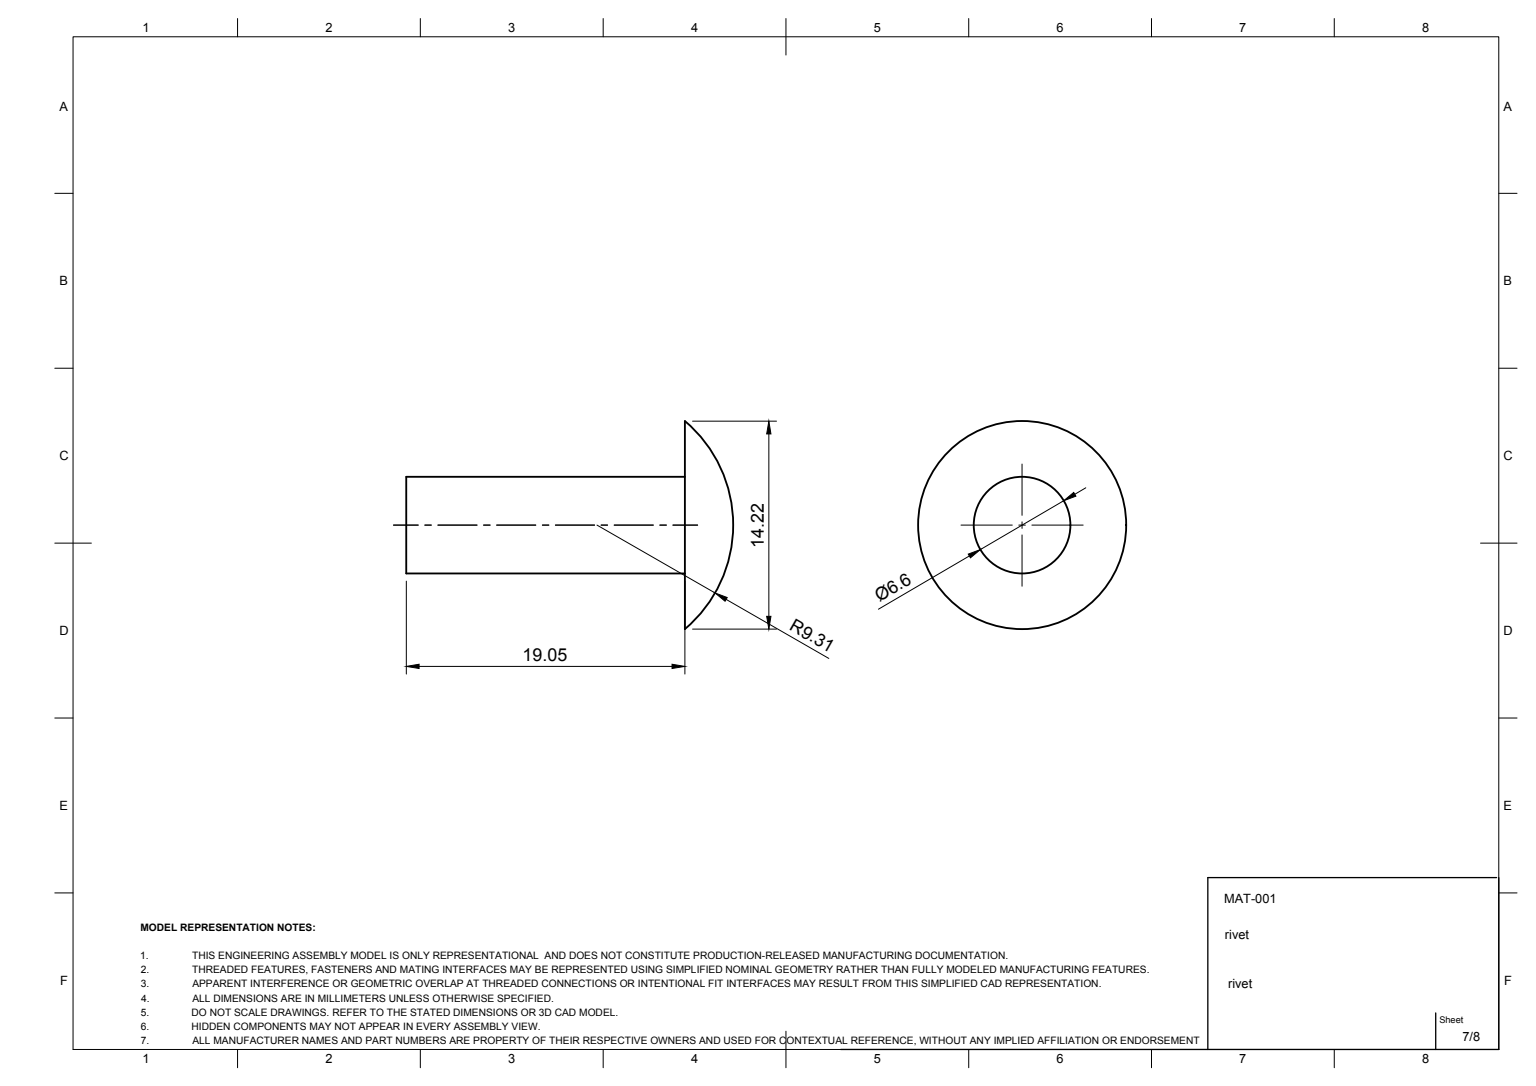
ISO-10303-21;
HEADER;
/* Generated by software containing ST-Developer
 * from STEP Tools, Inc. (www.steptools.com) 
 */

FILE_DESCRIPTION(
/* description */ ('STEP AP214'),
/* implementation_level */ '2;1');

FILE_NAME(
/* name */ 'Rivet.step',
/* time_stamp */ '2026-11-14T04:30:00-08:00',
/* author */ (''),
/* organization */ (''),
/* preprocessor_version */ 'ST-DEVELOPER v20.2',
/* originating_system */ 'Autodesk Translation Framework v15.17.0.0',
/* authorisation */ '');

FILE_SCHEMA (('AUTOMOTIVE_DESIGN { 1 0 10303 214 3 1 1 }'));
ENDSEC;

DATA;
#10=MECHANICAL_DESIGN_GEOMETRIC_PRESENTATION_REPRESENTATION('',(#127),#40809);
#111=SHAPE_REPRESENTATION_RELATIONSHIP('SRR','None',#40861,#119);
#119=ADVANCED_BREP_SHAPE_REPRESENTATION('',(#135),#40805);
#127=STYLED_ITEM('',(#40908),#135);
#135=MANIFOLD_SOLID_BREP('Body1',#6302);
#147=SPHERICAL_SURFACE('',#6832,9.31007692307692);
#296=PLANE('',#6834);
#297=PLANE('',#6835);
#353=FACE_BOUND('',#1147,.T.);
#742=FACE_OUTER_BOUND('',#1143,.T.);
#743=FACE_OUTER_BOUND('',#1144,.T.);
#744=FACE_OUTER_BOUND('',#1145,.T.);
#745=FACE_OUTER_BOUND('',#1146,.T.);
#1143=EDGE_LOOP('',(#5100,#5101,#5102,#5103));
#1144=EDGE_LOOP('',(#5104));
#1145=EDGE_LOOP('',(#5105));
#1146=EDGE_LOOP('',(#5106));
#1147=EDGE_LOOP('',(#5107));
#1512=CIRCLE('',#6830,3.302);
#1513=CIRCLE('',#6831,3.302);
#1514=CIRCLE('',#6833,7.11199999999999);
#2005=LINE('',#40023,#2323);
#2323=VECTOR('',#8235,3.302);
#2813=VERTEX_POINT('',#40020);
#2814=VERTEX_POINT('',#40022);
#2815=VERTEX_POINT('',#40026);
#3602=EDGE_CURVE('',#2813,#2813,#1512,.T.);
#3603=EDGE_CURVE('',#2813,#2814,#2005,.T.);
#3604=EDGE_CURVE('',#2814,#2814,#1513,.T.);
#3605=EDGE_CURVE('',#2815,#2815,#1514,.T.);
#5100=ORIENTED_EDGE('',*,*,#3602,.F.);
#5101=ORIENTED_EDGE('',*,*,#3603,.T.);
#5102=ORIENTED_EDGE('',*,*,#3604,.T.);
#5103=ORIENTED_EDGE('',*,*,#3603,.F.);
#5104=ORIENTED_EDGE('',*,*,#3605,.F.);
#5105=ORIENTED_EDGE('',*,*,#3602,.T.);
#5106=ORIENTED_EDGE('',*,*,#3605,.T.);
#5107=ORIENTED_EDGE('',*,*,#3604,.F.);
#5872=CYLINDRICAL_SURFACE('',#6829,3.302);
#6157=ADVANCED_FACE('',(#742),#5872,.T.);
#6158=ADVANCED_FACE('',(#743),#147,.T.);
#6159=ADVANCED_FACE('',(#744),#296,.T.);
#6160=ADVANCED_FACE('',(#745,#353),#297,.T.);
#6302=CLOSED_SHELL('',(#6157,#6158,#6159,#6160));
#6828=AXIS2_PLACEMENT_3D('',#40018,#8229,#8230);
#6829=AXIS2_PLACEMENT_3D('',#40019,#8231,#8232);
#6830=AXIS2_PLACEMENT_3D('',#40021,#8233,#8234);
#6831=AXIS2_PLACEMENT_3D('',#40024,#8236,#8237);
#6832=AXIS2_PLACEMENT_3D('',#40025,#8238,#8239);
#6833=AXIS2_PLACEMENT_3D('',#40027,#8240,#8241);
#6834=AXIS2_PLACEMENT_3D('',#40028,#8242,#8243);
#6835=AXIS2_PLACEMENT_3D('',#40029,#8244,#8245);
#8229=DIRECTION('axis',(0.,0.,1.));
#8230=DIRECTION('refdir',(1.,0.,0.));
#8231=DIRECTION('center_axis',(-8.48851915644968E-18,0.,-1.));
#8232=DIRECTION('ref_axis',(-1.,0.,8.48851915644968E-18));
#8233=DIRECTION('center_axis',(-8.48851915644968E-18,0.,-1.));
#8234=DIRECTION('ref_axis',(-1.,0.,8.48851915644968E-18));
#8235=DIRECTION('',(8.48851915644968E-18,0.,1.));
#8236=DIRECTION('center_axis',(-8.48851915644968E-18,0.,-1.));
#8237=DIRECTION('ref_axis',(-1.,0.,8.48851915644968E-18));
#8238=DIRECTION('center_axis',(-6.12323399573677E-17,1.,0.));
#8239=DIRECTION('ref_axis',(-1.,0.,0.));
#8240=DIRECTION('center_axis',(-8.48851915644968E-18,0.,-1.));
#8241=DIRECTION('ref_axis',(-1.,0.,8.48851915644968E-18));
#8242=DIRECTION('center_axis',(-8.48851915644968E-18,0.,-1.));
#8243=DIRECTION('ref_axis',(-1.,0.,8.48851915644968E-18));
#8244=DIRECTION('center_axis',(-8.48851915644968E-18,0.,-1.));
#8245=DIRECTION('ref_axis',(-1.,0.,8.48851915644968E-18));
#40018=CARTESIAN_POINT('',(0.,0.,0.));
#40019=CARTESIAN_POINT('Origin',(-1.89735380184963E-16,0.,-22.352));
#40020=CARTESIAN_POINT('',(3.302,-4.04378373078456E-16,-22.352));
#40021=CARTESIAN_POINT('Origin',(-1.89735380184963E-16,0.,-22.352));
#40022=CARTESIAN_POINT('',(3.302,-4.04378373078456E-16,-3.302));
#40023=CARTESIAN_POINT('',(3.302,-4.04378373078456E-16,-22.352));
#40024=CARTESIAN_POINT('Origin',(-2.80290902545968E-17,0.,-3.302));
#40025=CARTESIAN_POINT('Origin',(1.73472347597681E-15,0.,-9.31007692307692));
#40026=CARTESIAN_POINT('',(7.112,8.70968803553597E-16,-3.302));
#40027=CARTESIAN_POINT('Origin',(-2.80290902545968E-17,0.,-3.302));
#40028=CARTESIAN_POINT('Origin',(-3.302,0.,-22.352));
#40029=CARTESIAN_POINT('Origin',(-7.112,0.,-3.302));
#40795=UNCERTAINTY_MEASURE_WITH_UNIT(LENGTH_MEASURE(0.01),#40810,
'DISTANCE_ACCURACY_VALUE',
'Maximum model space distance between geometric entities at asserted c
onnectivities');
#40799=UNCERTAINTY_MEASURE_WITH_UNIT(LENGTH_MEASURE(0.01),#40810,
'DISTANCE_ACCURACY_VALUE',
'Maximum model space distance between geometric entities at asserted c
onnectivities');
#40805=(
GEOMETRIC_REPRESENTATION_CONTEXT(3)
GLOBAL_UNCERTAINTY_ASSIGNED_CONTEXT((#40795))
GLOBAL_UNIT_ASSIGNED_CONTEXT((#40810,#40812,#40813))
REPRESENTATION_CONTEXT('','3D')
);
#40809=(
GEOMETRIC_REPRESENTATION_CONTEXT(3)
GLOBAL_UNCERTAINTY_ASSIGNED_CONTEXT((#40799))
GLOBAL_UNIT_ASSIGNED_CONTEXT((#40810,#40812,#40813))
REPRESENTATION_CONTEXT('','3D')
);
#40810=(
LENGTH_UNIT()
NAMED_UNIT(*)
SI_UNIT(.MILLI.,.METRE.)
);
#40812=(
NAMED_UNIT(*)
PLANE_ANGLE_UNIT()
SI_UNIT($,.RADIAN.)
);
#40813=(
NAMED_UNIT(*)
SI_UNIT($,.STERADIAN.)
SOLID_ANGLE_UNIT()
);
#40819=SHAPE_DEFINITION_REPRESENTATION(#40828,#40861);
#40828=PRODUCT_DEFINITION_SHAPE('',$,#40871);
#40861=SHAPE_REPRESENTATION('',(#6828),#40805);
#40865=PRODUCT_DEFINITION_CONTEXT('part definition',#40894,'design');
#40871=PRODUCT_DEFINITION('rivet','Rivet',#40880,#40865);
#40880=PRODUCT_DEFINITION_FORMATION('',$,#40901);
#40894=APPLICATION_CONTEXT(
'Core Data for Automotive Mechanical Design Process');
#40895=PRODUCT_CONTEXT('part definition',#40894,'mechanical');
#40901=PRODUCT('rivet','Rivet',$,(#40895));
#40908=PRESENTATION_STYLE_ASSIGNMENT((#40913));
#40913=SURFACE_STYLE_USAGE(.BOTH.,#40918);
#40918=SURFACE_SIDE_STYLE('',(#40923));
#40923=SURFACE_STYLE_FILL_AREA(#40928);
#40928=FILL_AREA_STYLE('Opaque(61,176,222)',(#40933));
#40933=FILL_AREA_STYLE_COLOUR('Opaque(61,176,222)',#40938);
#40938=COLOUR_RGB('Opaque(61,176,222)',0.23921568627451,0.690196078431373,
0.870588235294118);
ENDSEC;
END-ISO-10303-21;
